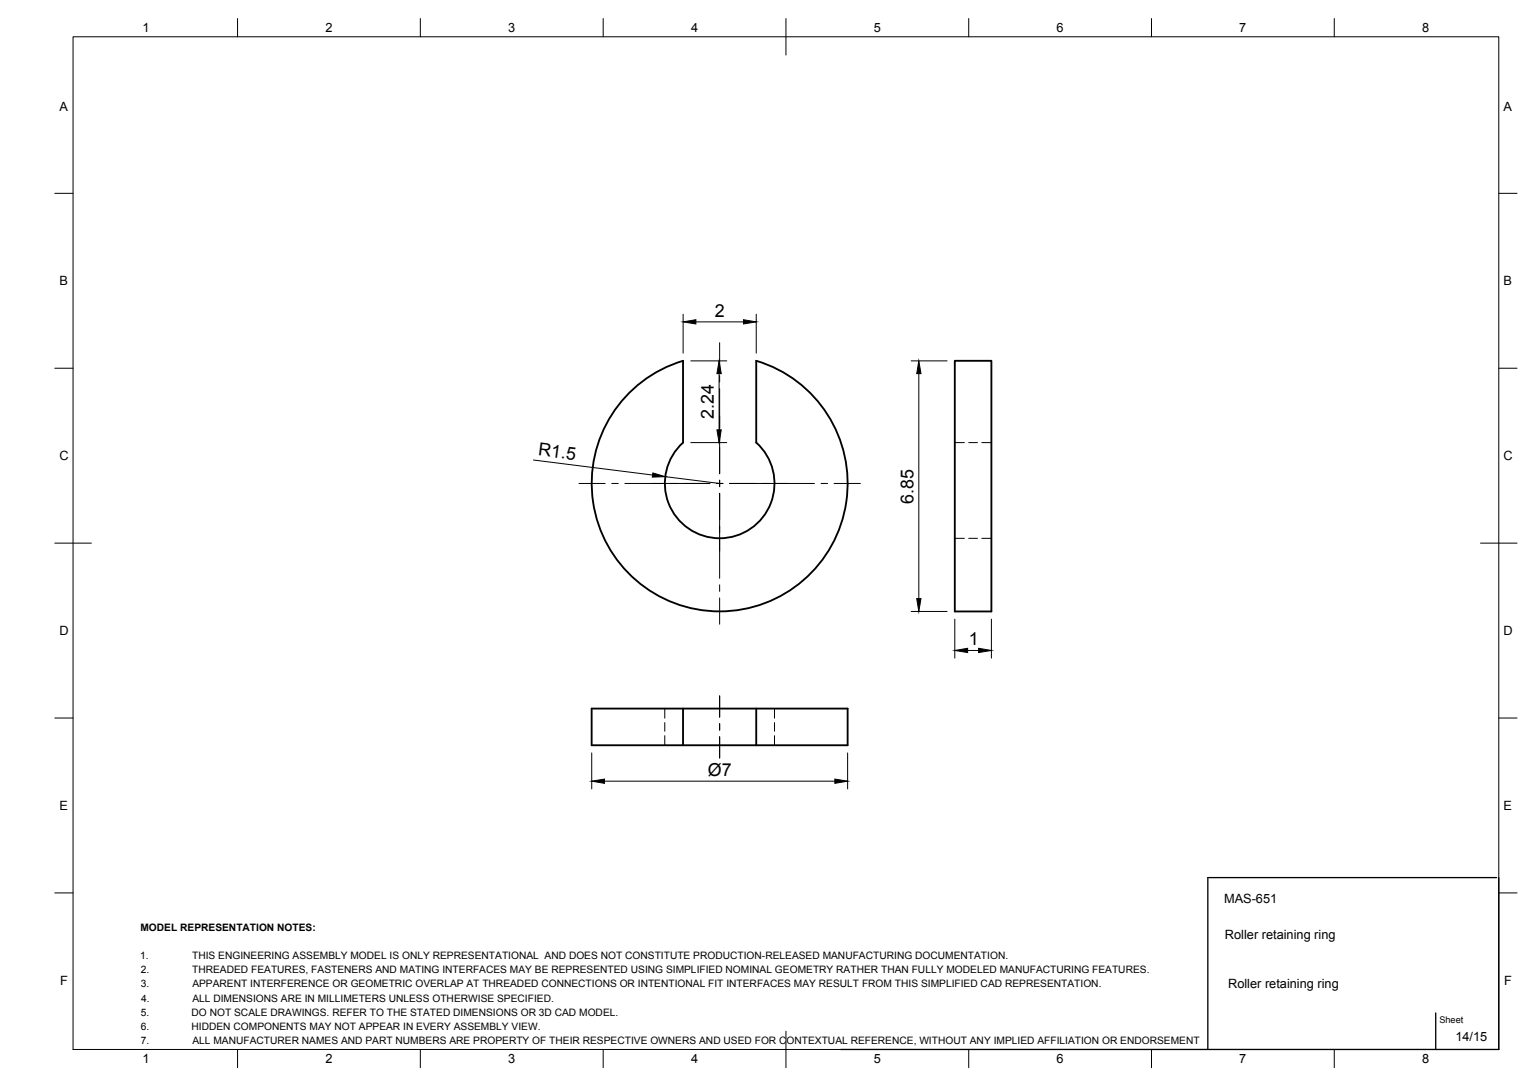
ISO-10303-21;
HEADER;
/* Generated by software containing ST-Developer
 * from STEP Tools, Inc. (www.steptools.com) 
 */

FILE_DESCRIPTION(
/* description */ ('Independent direct-acting normally-closed roller-plunger limit-switch
 CAD. Removable cover, insulated terminal supports, captured bus/conta
ct bridge, native Coil return spring, integral lower travel stop, reus
able instanced hardware and free roller. Manual geometric contact open
ing4mm; no snap-action/contact-force, electrical/current/voltage, envi
ronmental seal, safety-switch, wear, load or life certification. Exter
nal wiring and anchors omitted; fits and application engineering requi
red.'),
/* implementation_level */ '2;1');

FILE_NAME(
/* name */ 'Roller retaining ring.step',
/* time_stamp */ '2026-11-08T07:32:43-08:00',
/* author */ (''),
/* organization */ (''),
/* preprocessor_version */ 'ST-DEVELOPER v20.2',
/* originating_system */ 'Autodesk Translation Framework v15.17.0.0',
/* authorisation */ '');

FILE_SCHEMA (('AUTOMOTIVE_DESIGN { 1 0 10303 214 3 1 1 }'));
ENDSEC;

DATA;
#10=MECHANICAL_DESIGN_GEOMETRIC_PRESENTATION_REPRESENTATION('',(#187),#36482);
#153=SHAPE_REPRESENTATION_RELATIONSHIP('SRR','None',#36566,#170);
#170=ADVANCED_BREP_SHAPE_REPRESENTATION('',(#204),#36476);
#187=STYLED_ITEM('',(#36659),#204);
#204=MANIFOLD_SOLID_BREP('Body1',#9778);
#401=PLANE('',#10481);
#402=PLANE('',#10482);
#403=PLANE('',#10483);
#404=PLANE('',#10490);
#828=FACE_OUTER_BOUND('',#1425,.T.);
#829=FACE_OUTER_BOUND('',#1426,.T.);
#830=FACE_OUTER_BOUND('',#1427,.T.);
#831=FACE_OUTER_BOUND('',#1428,.T.);
#832=FACE_OUTER_BOUND('',#1429,.T.);
#833=FACE_OUTER_BOUND('',#1430,.T.);
#1425=EDGE_LOOP('',(#8074,#8075,#8076,#8077));
#1426=EDGE_LOOP('',(#8078,#8079,#8080,#8081));
#1427=EDGE_LOOP('',(#8082,#8083,#8084,#8085));
#1428=EDGE_LOOP('',(#8086,#8087,#8088,#8089));
#1429=EDGE_LOOP('',(#8090,#8091,#8092,#8093));
#1430=EDGE_LOOP('',(#8094,#8095,#8096,#8097));
#1707=CIRCLE('',#10484,0.35);
#1708=CIRCLE('',#10485,0.15);
#1709=CIRCLE('',#10487,0.15);
#1710=CIRCLE('',#10489,0.35);
#2861=LINE('',#29291,#3435);
#2862=LINE('',#29293,#3436);
#2863=LINE('',#29295,#3437);
#2864=LINE('',#29296,#3438);
#2865=LINE('',#29300,#3439);
#2866=LINE('',#29302,#3440);
#2867=LINE('',#29304,#3441);
#2868=LINE('',#29305,#3442);
#3435=VECTOR('',#12126,1.);
#3436=VECTOR('',#12127,1.);
#3437=VECTOR('',#12128,1.);
#3438=VECTOR('',#12129,1.);
#3439=VECTOR('',#12132,1.);
#3440=VECTOR('',#12133,1.);
#3441=VECTOR('',#12134,1.);
#3442=VECTOR('',#12135,1.);
#4287=VERTEX_POINT('',#29289);
#4288=VERTEX_POINT('',#29290);
#4289=VERTEX_POINT('',#29292);
#4290=VERTEX_POINT('',#29294);
#4291=VERTEX_POINT('',#29298);
#4292=VERTEX_POINT('',#29299);
#4293=VERTEX_POINT('',#29301);
#4294=VERTEX_POINT('',#29303);
#5593=EDGE_CURVE('',#4287,#4288,#2861,.T.);
#5594=EDGE_CURVE('',#4289,#4287,#2862,.T.);
#5595=EDGE_CURVE('',#4290,#4289,#2863,.T.);
#5596=EDGE_CURVE('',#4288,#4290,#2864,.T.);
#5597=EDGE_CURVE('',#4291,#4292,#2865,.T.);
#5598=EDGE_CURVE('',#4293,#4291,#2866,.T.);
#5599=EDGE_CURVE('',#4294,#4293,#2867,.T.);
#5600=EDGE_CURVE('',#4292,#4294,#2868,.T.);
#5601=EDGE_CURVE('',#4289,#4294,#1707,.T.);
#5602=EDGE_CURVE('',#4292,#4287,#1708,.T.);
#5603=EDGE_CURVE('',#4291,#4288,#1709,.T.);
#5604=EDGE_CURVE('',#4290,#4293,#1710,.T.);
#8074=ORIENTED_EDGE('',*,*,#5593,.F.);
#8075=ORIENTED_EDGE('',*,*,#5594,.F.);
#8076=ORIENTED_EDGE('',*,*,#5595,.F.);
#8077=ORIENTED_EDGE('',*,*,#5596,.F.);
#8078=ORIENTED_EDGE('',*,*,#5597,.F.);
#8079=ORIENTED_EDGE('',*,*,#5598,.F.);
#8080=ORIENTED_EDGE('',*,*,#5599,.F.);
#8081=ORIENTED_EDGE('',*,*,#5600,.F.);
#8082=ORIENTED_EDGE('',*,*,#5600,.T.);
#8083=ORIENTED_EDGE('',*,*,#5601,.F.);
#8084=ORIENTED_EDGE('',*,*,#5594,.T.);
#8085=ORIENTED_EDGE('',*,*,#5602,.F.);
#8086=ORIENTED_EDGE('',*,*,#5597,.T.);
#8087=ORIENTED_EDGE('',*,*,#5602,.T.);
#8088=ORIENTED_EDGE('',*,*,#5593,.T.);
#8089=ORIENTED_EDGE('',*,*,#5603,.F.);
#8090=ORIENTED_EDGE('',*,*,#5599,.T.);
#8091=ORIENTED_EDGE('',*,*,#5604,.F.);
#8092=ORIENTED_EDGE('',*,*,#5595,.T.);
#8093=ORIENTED_EDGE('',*,*,#5601,.T.);
#8094=ORIENTED_EDGE('',*,*,#5598,.T.);
#8095=ORIENTED_EDGE('',*,*,#5603,.T.);
#8096=ORIENTED_EDGE('',*,*,#5596,.T.);
#8097=ORIENTED_EDGE('',*,*,#5604,.T.);
#9128=CYLINDRICAL_SURFACE('',#10486,0.15);
#9129=CYLINDRICAL_SURFACE('',#10488,0.35);
#9618=ADVANCED_FACE('',(#828),#401,.F.);
#9619=ADVANCED_FACE('',(#829),#402,.F.);
#9620=ADVANCED_FACE('',(#830),#403,.F.);
#9621=ADVANCED_FACE('',(#831),#9128,.F.);
#9622=ADVANCED_FACE('',(#832),#9129,.T.);
#9623=ADVANCED_FACE('',(#833),#404,.T.);
#9778=CLOSED_SHELL('',(#9618,#9619,#9620,#9621,#9622,#9623));
#10480=AXIS2_PLACEMENT_3D('',#29287,#12122,#12123);
#10481=AXIS2_PLACEMENT_3D('',#29288,#12124,#12125);
#10482=AXIS2_PLACEMENT_3D('',#29297,#12130,#12131);
#10483=AXIS2_PLACEMENT_3D('',#29306,#12136,#12137);
#10484=AXIS2_PLACEMENT_3D('',#29307,#12138,#12139);
#10485=AXIS2_PLACEMENT_3D('',#29308,#12140,#12141);
#10486=AXIS2_PLACEMENT_3D('',#29309,#12142,#12143);
#10487=AXIS2_PLACEMENT_3D('',#29310,#12144,#12145);
#10488=AXIS2_PLACEMENT_3D('',#29311,#12146,#12147);
#10489=AXIS2_PLACEMENT_3D('',#29312,#12148,#12149);
#10490=AXIS2_PLACEMENT_3D('',#29313,#12150,#12151);
#12122=DIRECTION('axis',(0.,0.,1.));
#12123=DIRECTION('refdir',(1.,0.,0.));
#12124=DIRECTION('center_axis',(-1.,0.,0.));
#12125=DIRECTION('ref_axis',(0.,1.,0.));
#12126=DIRECTION('',(0.,0.,1.));
#12127=DIRECTION('',(0.,-1.,0.));
#12128=DIRECTION('',(0.,0.,-1.));
#12129=DIRECTION('',(0.,1.,0.));
#12130=DIRECTION('center_axis',(1.,0.,0.));
#12131=DIRECTION('ref_axis',(0.,-1.,0.));
#12132=DIRECTION('',(0.,0.,-1.));
#12133=DIRECTION('',(0.,-1.,0.));
#12134=DIRECTION('',(0.,0.,1.));
#12135=DIRECTION('',(0.,1.,0.));
#12136=DIRECTION('center_axis',(0.,0.,1.));
#12137=DIRECTION('ref_axis',(1.,0.,0.));
#12138=DIRECTION('center_axis',(0.,0.,1.));
#12139=DIRECTION('ref_axis',(1.,0.,0.));
#12140=DIRECTION('center_axis',(0.,0.,-1.));
#12141=DIRECTION('ref_axis',(1.,0.,0.));
#12142=DIRECTION('center_axis',(0.,0.,1.));
#12143=DIRECTION('ref_axis',(6.12323399573677E-17,-1.,0.));
#12144=DIRECTION('center_axis',(0.,0.,-1.));
#12145=DIRECTION('ref_axis',(1.,0.,0.));
#12146=DIRECTION('center_axis',(0.,0.,1.));
#12147=DIRECTION('ref_axis',(6.12323399573677E-17,-1.,0.));
#12148=DIRECTION('center_axis',(0.,0.,1.));
#12149=DIRECTION('ref_axis',(1.,0.,0.));
#12150=DIRECTION('center_axis',(0.,0.,1.));
#12151=DIRECTION('ref_axis',(1.,0.,0.));
#29287=CARTESIAN_POINT('',(0.,0.,0.));
#29288=CARTESIAN_POINT('Origin',(-0.1,0.,0.1));
#29289=CARTESIAN_POINT('',(-0.1,0.111803398874989,0.));
#29290=CARTESIAN_POINT('',(-0.1,0.111803398874989,0.1));
#29291=CARTESIAN_POINT('',(-0.1,0.111803398874989,0.));
#29292=CARTESIAN_POINT('',(-0.1,0.335410196624968,0.));
#29293=CARTESIAN_POINT('',(-0.1,0.,0.));
#29294=CARTESIAN_POINT('',(-0.1,0.335410196624968,0.1));
#29295=CARTESIAN_POINT('',(-0.1,0.335410196624968,0.));
#29296=CARTESIAN_POINT('',(-0.1,0.,0.1));
#29297=CARTESIAN_POINT('Origin',(0.1,0.7,0.1));
#29298=CARTESIAN_POINT('',(0.1,0.111803398874989,0.1));
#29299=CARTESIAN_POINT('',(0.1,0.111803398874989,0.));
#29300=CARTESIAN_POINT('',(0.1,0.111803398874989,0.));
#29301=CARTESIAN_POINT('',(0.1,0.335410196624968,0.1));
#29302=CARTESIAN_POINT('',(0.1,0.35,0.1));
#29303=CARTESIAN_POINT('',(0.1,0.335410196624968,0.));
#29304=CARTESIAN_POINT('',(0.1,0.335410196624968,0.));
#29305=CARTESIAN_POINT('',(0.1,0.35,0.));
#29306=CARTESIAN_POINT('Origin',(0.,0.,0.));
#29307=CARTESIAN_POINT('Origin',(0.,0.,0.));
#29308=CARTESIAN_POINT('Origin',(0.,0.,0.));
#29309=CARTESIAN_POINT('Origin',(0.,0.,0.));
#29310=CARTESIAN_POINT('Origin',(0.,0.,0.1));
#29311=CARTESIAN_POINT('Origin',(0.,0.,0.));
#29312=CARTESIAN_POINT('Origin',(0.,0.,0.1));
#29313=CARTESIAN_POINT('Origin',(0.,0.,0.1));
#36457=UNCERTAINTY_MEASURE_WITH_UNIT(LENGTH_MEASURE(0.001),#36483,
'DISTANCE_ACCURACY_VALUE',
'Maximum model space distance between geometric entities at asserted c
onnectivities');
#36463=UNCERTAINTY_MEASURE_WITH_UNIT(LENGTH_MEASURE(0.001),#36483,
'DISTANCE_ACCURACY_VALUE',
'Maximum model space distance between geometric entities at asserted c
onnectivities');
#36476=(
GEOMETRIC_REPRESENTATION_CONTEXT(3)
GLOBAL_UNCERTAINTY_ASSIGNED_CONTEXT((#36457))
GLOBAL_UNIT_ASSIGNED_CONTEXT((#36483,#36485,#36486))
REPRESENTATION_CONTEXT('','3D')
);
#36482=(
GEOMETRIC_REPRESENTATION_CONTEXT(3)
GLOBAL_UNCERTAINTY_ASSIGNED_CONTEXT((#36463))
GLOBAL_UNIT_ASSIGNED_CONTEXT((#36483,#36485,#36486))
REPRESENTATION_CONTEXT('','3D')
);
#36483=(
LENGTH_UNIT()
NAMED_UNIT(*)
SI_UNIT(.CENTI.,.METRE.)
);
#36485=(
NAMED_UNIT(*)
PLANE_ANGLE_UNIT()
SI_UNIT($,.RADIAN.)
);
#36486=(
NAMED_UNIT(*)
SI_UNIT($,.STERADIAN.)
SOLID_ANGLE_UNIT()
);
#36499=SHAPE_DEFINITION_REPRESENTATION(#36517,#36566);
#36517=PRODUCT_DEFINITION_SHAPE('',$,#36585);
#36566=SHAPE_REPRESENTATION('',(#10480),#36476);
#36572=PRODUCT_DEFINITION_CONTEXT('part definition',#36628,'design');
#36585=PRODUCT_DEFINITION('Roller retaining ring',
'Roller retaining ring',#36603,#36572);
#36603=PRODUCT_DEFINITION_FORMATION('',$,#36642);
#36628=APPLICATION_CONTEXT(
'Core Data for Automotive Mechanical Design Process');
#36629=PRODUCT_CONTEXT('part definition',#36628,'mechanical');
#36642=PRODUCT('Roller retaining ring','Roller retaining ring',$,(#36629));
#36659=PRESENTATION_STYLE_ASSIGNMENT((#36673));
#36673=SURFACE_STYLE_USAGE(.BOTH.,#36687);
#36687=SURFACE_SIDE_STYLE('',(#36701));
#36701=SURFACE_STYLE_FILL_AREA(#36715);
#36715=FILL_AREA_STYLE('Dark gray',(#36729));
#36729=FILL_AREA_STYLE_COLOUR('Dark gray',#36743);
#36743=COLOUR_RGB('Dark gray',0.250980392156863,0.282352941176471,0.32156862745098);
ENDSEC;
END-ISO-10303-21;
